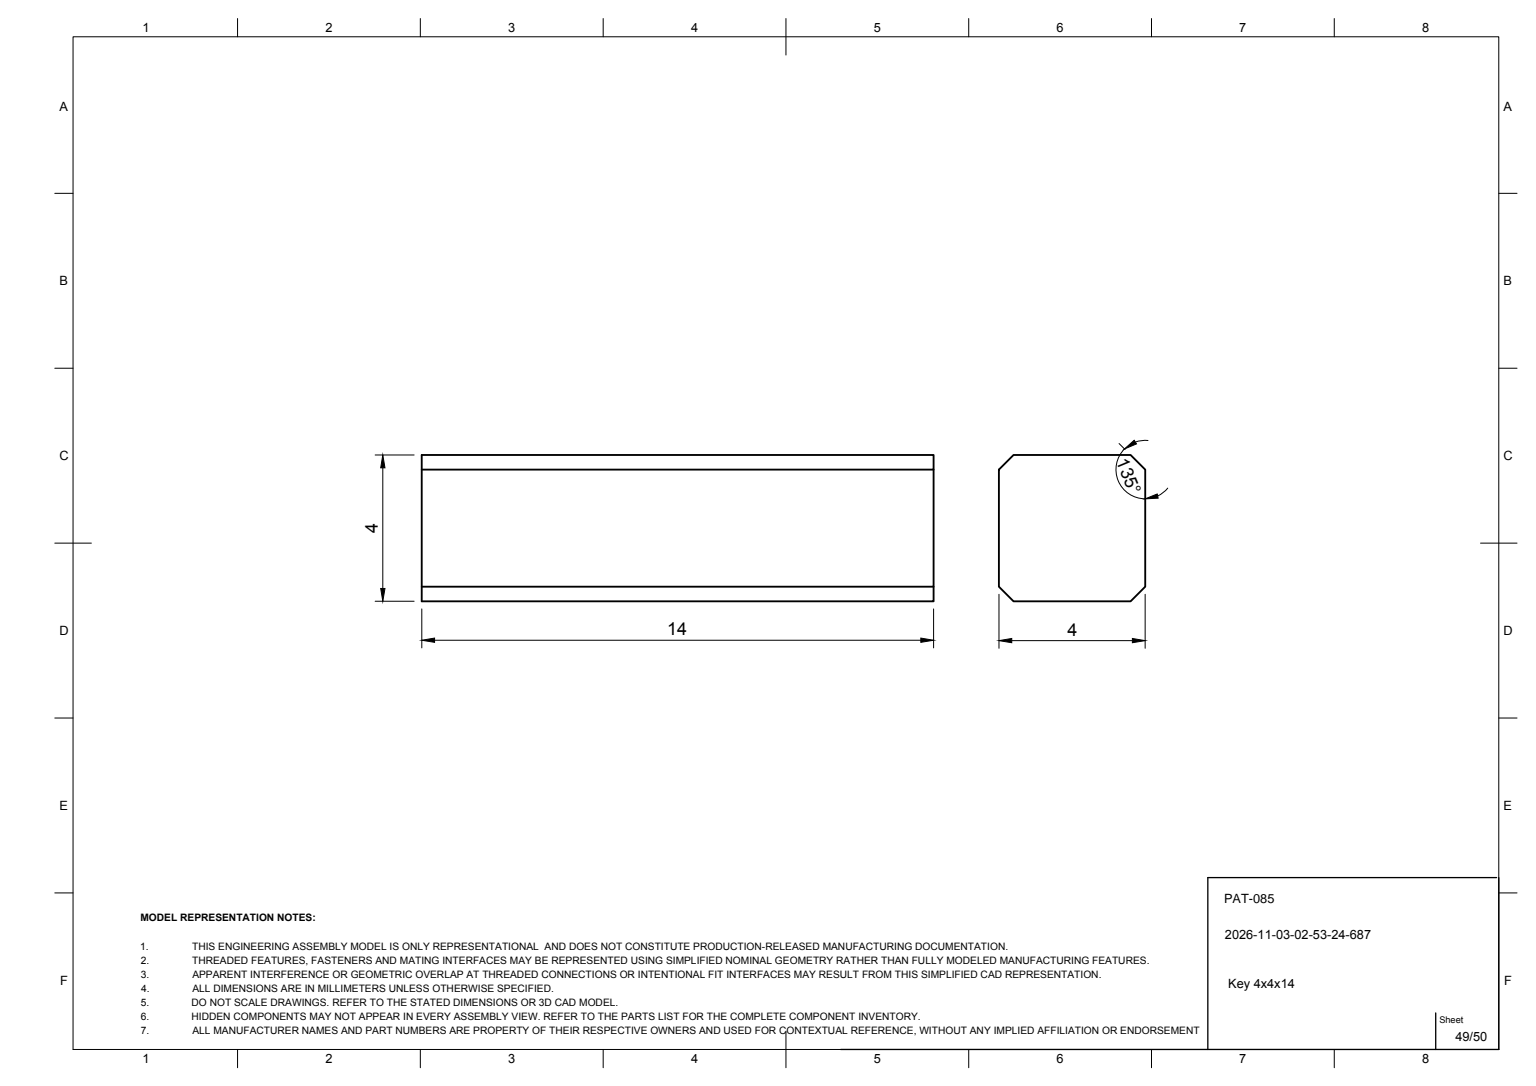
ISO-10303-21;
HEADER;
/* Generated by software containing ST-Developer
 * from STEP Tools, Inc. (www.steptools.com) 
 */

FILE_DESCRIPTION(
/* description */ ('Rack and pinion manual slide'),
/* implementation_level */ '2;1');

FILE_NAME(
/* name */ 'Key 4x4x14.step',
/* time_stamp */ '2026-10-28T03:22:49-07:00',
/* author */ (''),
/* organization */ (''),
/* preprocessor_version */ 'ST-DEVELOPER v20.2',
/* originating_system */ 'Autodesk Translation Framework v15.17.0.0',
/* authorisation */ '');

FILE_SCHEMA (('AUTOMOTIVE_DESIGN { 1 0 10303 214 3 1 1 }'));
ENDSEC;

DATA;
#10=MECHANICAL_DESIGN_GEOMETRIC_PRESENTATION_REPRESENTATION('',(#781),#34851);
#682=SHAPE_REPRESENTATION_RELATIONSHIP('SRR','None',#35121,#728);
#728=ADVANCED_BREP_SHAPE_REPRESENTATION('',(#830),#34846);
#781=STYLED_ITEM('',(#35411),#830);
#830=MANIFOLD_SOLID_BREP('Body1',#13805);
#1510=PLANE('',#15524);
#1511=PLANE('',#15525);
#1512=PLANE('',#15526);
#1513=PLANE('',#15527);
#1514=PLANE('',#15528);
#1515=PLANE('',#15529);
#1516=PLANE('',#15530);
#1517=PLANE('',#15531);
#1518=PLANE('',#15532);
#1519=PLANE('',#15533);
#2239=FACE_OUTER_BOUND('',#3184,.T.);
#2240=FACE_OUTER_BOUND('',#3185,.T.);
#2241=FACE_OUTER_BOUND('',#3186,.T.);
#2242=FACE_OUTER_BOUND('',#3187,.T.);
#2243=FACE_OUTER_BOUND('',#3188,.T.);
#2244=FACE_OUTER_BOUND('',#3189,.T.);
#2245=FACE_OUTER_BOUND('',#3190,.T.);
#2246=FACE_OUTER_BOUND('',#3191,.T.);
#2247=FACE_OUTER_BOUND('',#3192,.T.);
#2248=FACE_OUTER_BOUND('',#3193,.T.);
#3184=EDGE_LOOP('',(#12708,#12709,#12710,#12711,#12712,#12713,#12714,#12715));
#3185=EDGE_LOOP('',(#12716,#12717,#12718,#12719));
#3186=EDGE_LOOP('',(#12720,#12721,#12722,#12723));
#3187=EDGE_LOOP('',(#12724,#12725,#12726,#12727));
#3188=EDGE_LOOP('',(#12728,#12729,#12730,#12731));
#3189=EDGE_LOOP('',(#12732,#12733,#12734,#12735,#12736,#12737,#12738,#12739));
#3190=EDGE_LOOP('',(#12740,#12741,#12742,#12743));
#3191=EDGE_LOOP('',(#12744,#12745,#12746,#12747));
#3192=EDGE_LOOP('',(#12748,#12749,#12750,#12751));
#3193=EDGE_LOOP('',(#12752,#12753,#12754,#12755));
#4463=LINE('',#34575,#5754);
#4464=LINE('',#34577,#5755);
#4465=LINE('',#34579,#5756);
#4466=LINE('',#34581,#5757);
#4467=LINE('',#34583,#5758);
#4468=LINE('',#34585,#5759);
#4469=LINE('',#34587,#5760);
#4470=LINE('',#34588,#5761);
#4471=LINE('',#34591,#5762);
#4472=LINE('',#34593,#5763);
#4473=LINE('',#34594,#5764);
#4474=LINE('',#34597,#5765);
#4475=LINE('',#34598,#5766);
#4476=LINE('',#34601,#5767);
#4477=LINE('',#34602,#5768);
#4478=LINE('',#34605,#5769);
#4479=LINE('',#34606,#5770);
#4480=LINE('',#34609,#5771);
#4481=LINE('',#34611,#5772);
#4482=LINE('',#34613,#5773);
#4483=LINE('',#34614,#5774);
#4484=LINE('',#34616,#5775);
#4485=LINE('',#34618,#5776);
#4486=LINE('',#34620,#5777);
#5754=VECTOR('',#19255,1.);
#5755=VECTOR('',#19256,1.);
#5756=VECTOR('',#19257,1.);
#5757=VECTOR('',#19258,1.);
#5758=VECTOR('',#19259,1.);
#5759=VECTOR('',#19260,1.);
#5760=VECTOR('',#19261,1.);
#5761=VECTOR('',#19262,1.);
#5762=VECTOR('',#19265,1.);
#5763=VECTOR('',#19266,1.);
#5764=VECTOR('',#19267,1.);
#5765=VECTOR('',#19270,1.);
#5766=VECTOR('',#19271,1.);
#5767=VECTOR('',#19274,1.);
#5768=VECTOR('',#19275,1.);
#5769=VECTOR('',#19278,1.);
#5770=VECTOR('',#19279,1.);
#5771=VECTOR('',#19282,1.);
#5772=VECTOR('',#19283,1.);
#5773=VECTOR('',#19284,1.);
#5774=VECTOR('',#19285,1.);
#5775=VECTOR('',#19288,1.);
#5776=VECTOR('',#19291,1.);
#5777=VECTOR('',#19294,1.);
#7385=VERTEX_POINT('',#34573);
#7386=VERTEX_POINT('',#34574);
#7387=VERTEX_POINT('',#34576);
#7388=VERTEX_POINT('',#34578);
#7389=VERTEX_POINT('',#34580);
#7390=VERTEX_POINT('',#34582);
#7391=VERTEX_POINT('',#34584);
#7392=VERTEX_POINT('',#34586);
#7393=VERTEX_POINT('',#34590);
#7394=VERTEX_POINT('',#34592);
#7395=VERTEX_POINT('',#34596);
#7396=VERTEX_POINT('',#34600);
#7397=VERTEX_POINT('',#34604);
#7398=VERTEX_POINT('',#34608);
#7399=VERTEX_POINT('',#34610);
#7400=VERTEX_POINT('',#34612);
#9166=EDGE_CURVE('',#7385,#7386,#4463,.T.);
#9167=EDGE_CURVE('',#7387,#7385,#4464,.T.);
#9168=EDGE_CURVE('',#7388,#7387,#4465,.T.);
#9169=EDGE_CURVE('',#7389,#7388,#4466,.T.);
#9170=EDGE_CURVE('',#7390,#7389,#4467,.T.);
#9171=EDGE_CURVE('',#7391,#7390,#4468,.T.);
#9172=EDGE_CURVE('',#7392,#7391,#4469,.T.);
#9173=EDGE_CURVE('',#7386,#7392,#4470,.T.);
#9174=EDGE_CURVE('',#7389,#7393,#4471,.T.);
#9175=EDGE_CURVE('',#7393,#7394,#4472,.T.);
#9176=EDGE_CURVE('',#7394,#7390,#4473,.T.);
#9177=EDGE_CURVE('',#7395,#7388,#4474,.T.);
#9178=EDGE_CURVE('',#7395,#7393,#4475,.T.);
#9179=EDGE_CURVE('',#7387,#7396,#4476,.T.);
#9180=EDGE_CURVE('',#7396,#7395,#4477,.T.);
#9181=EDGE_CURVE('',#7397,#7385,#4478,.T.);
#9182=EDGE_CURVE('',#7397,#7396,#4479,.T.);
#9183=EDGE_CURVE('',#7398,#7397,#4480,.T.);
#9184=EDGE_CURVE('',#7399,#7398,#4481,.T.);
#9185=EDGE_CURVE('',#7400,#7399,#4482,.T.);
#9186=EDGE_CURVE('',#7394,#7400,#4483,.T.);
#9187=EDGE_CURVE('',#7386,#7398,#4484,.T.);
#9188=EDGE_CURVE('',#7399,#7392,#4485,.T.);
#9189=EDGE_CURVE('',#7391,#7400,#4486,.T.);
#12708=ORIENTED_EDGE('',*,*,#9166,.F.);
#12709=ORIENTED_EDGE('',*,*,#9167,.F.);
#12710=ORIENTED_EDGE('',*,*,#9168,.F.);
#12711=ORIENTED_EDGE('',*,*,#9169,.F.);
#12712=ORIENTED_EDGE('',*,*,#9170,.F.);
#12713=ORIENTED_EDGE('',*,*,#9171,.F.);
#12714=ORIENTED_EDGE('',*,*,#9172,.F.);
#12715=ORIENTED_EDGE('',*,*,#9173,.F.);
#12716=ORIENTED_EDGE('',*,*,#9170,.T.);
#12717=ORIENTED_EDGE('',*,*,#9174,.T.);
#12718=ORIENTED_EDGE('',*,*,#9175,.T.);
#12719=ORIENTED_EDGE('',*,*,#9176,.T.);
#12720=ORIENTED_EDGE('',*,*,#9169,.T.);
#12721=ORIENTED_EDGE('',*,*,#9177,.F.);
#12722=ORIENTED_EDGE('',*,*,#9178,.T.);
#12723=ORIENTED_EDGE('',*,*,#9174,.F.);
#12724=ORIENTED_EDGE('',*,*,#9168,.T.);
#12725=ORIENTED_EDGE('',*,*,#9179,.T.);
#12726=ORIENTED_EDGE('',*,*,#9180,.T.);
#12727=ORIENTED_EDGE('',*,*,#9177,.T.);
#12728=ORIENTED_EDGE('',*,*,#9167,.T.);
#12729=ORIENTED_EDGE('',*,*,#9181,.F.);
#12730=ORIENTED_EDGE('',*,*,#9182,.T.);
#12731=ORIENTED_EDGE('',*,*,#9179,.F.);
#12732=ORIENTED_EDGE('',*,*,#9175,.F.);
#12733=ORIENTED_EDGE('',*,*,#9178,.F.);
#12734=ORIENTED_EDGE('',*,*,#9180,.F.);
#12735=ORIENTED_EDGE('',*,*,#9182,.F.);
#12736=ORIENTED_EDGE('',*,*,#9183,.F.);
#12737=ORIENTED_EDGE('',*,*,#9184,.F.);
#12738=ORIENTED_EDGE('',*,*,#9185,.F.);
#12739=ORIENTED_EDGE('',*,*,#9186,.F.);
#12740=ORIENTED_EDGE('',*,*,#9166,.T.);
#12741=ORIENTED_EDGE('',*,*,#9187,.T.);
#12742=ORIENTED_EDGE('',*,*,#9183,.T.);
#12743=ORIENTED_EDGE('',*,*,#9181,.T.);
#12744=ORIENTED_EDGE('',*,*,#9173,.T.);
#12745=ORIENTED_EDGE('',*,*,#9188,.F.);
#12746=ORIENTED_EDGE('',*,*,#9184,.T.);
#12747=ORIENTED_EDGE('',*,*,#9187,.F.);
#12748=ORIENTED_EDGE('',*,*,#9172,.T.);
#12749=ORIENTED_EDGE('',*,*,#9189,.T.);
#12750=ORIENTED_EDGE('',*,*,#9185,.T.);
#12751=ORIENTED_EDGE('',*,*,#9188,.T.);
#12752=ORIENTED_EDGE('',*,*,#9171,.T.);
#12753=ORIENTED_EDGE('',*,*,#9176,.F.);
#12754=ORIENTED_EDGE('',*,*,#9186,.T.);
#12755=ORIENTED_EDGE('',*,*,#9189,.F.);
#13717=ADVANCED_FACE('',(#2239),#1510,.T.);
#13718=ADVANCED_FACE('',(#2240),#1511,.T.);
#13719=ADVANCED_FACE('',(#2241),#1512,.T.);
#13720=ADVANCED_FACE('',(#2242),#1513,.T.);
#13721=ADVANCED_FACE('',(#2243),#1514,.T.);
#13722=ADVANCED_FACE('',(#2244),#1515,.F.);
#13723=ADVANCED_FACE('',(#2245),#1516,.T.);
#13724=ADVANCED_FACE('',(#2246),#1517,.T.);
#13725=ADVANCED_FACE('',(#2247),#1518,.T.);
#13726=ADVANCED_FACE('',(#2248),#1519,.F.);
#13805=CLOSED_SHELL('',(#13717,#13718,#13719,#13720,#13721,#13722,#13723,
#13724,#13725,#13726));
#15523=AXIS2_PLACEMENT_3D('',#34571,#19251,#19252);
#15524=AXIS2_PLACEMENT_3D('',#34572,#19253,#19254);
#15525=AXIS2_PLACEMENT_3D('',#34589,#19263,#19264);
#15526=AXIS2_PLACEMENT_3D('',#34595,#19268,#19269);
#15527=AXIS2_PLACEMENT_3D('',#34599,#19272,#19273);
#15528=AXIS2_PLACEMENT_3D('',#34603,#19276,#19277);
#15529=AXIS2_PLACEMENT_3D('',#34607,#19280,#19281);
#15530=AXIS2_PLACEMENT_3D('',#34615,#19286,#19287);
#15531=AXIS2_PLACEMENT_3D('',#34617,#19289,#19290);
#15532=AXIS2_PLACEMENT_3D('',#34619,#19292,#19293);
#15533=AXIS2_PLACEMENT_3D('',#34621,#19295,#19296);
#19251=DIRECTION('axis',(0.,0.,1.));
#19252=DIRECTION('refdir',(1.,0.,0.));
#19253=DIRECTION('center_axis',(1.,0.,0.));
#19254=DIRECTION('ref_axis',(0.,0.,-1.));
#19255=DIRECTION('',(0.,0.707106781186547,-0.707106781186548));
#19256=DIRECTION('',(0.,1.,0.));
#19257=DIRECTION('',(0.,0.707106781186547,0.707106781186548));
#19258=DIRECTION('',(0.,0.,1.));
#19259=DIRECTION('',(0.,-0.707106781186548,0.707106781186548));
#19260=DIRECTION('',(0.,-1.,0.));
#19261=DIRECTION('',(0.,-0.707106781186548,-0.707106781186548));
#19262=DIRECTION('',(0.,0.,-1.));
#19263=DIRECTION('center_axis',(0.,-0.707106781186548,-0.707106781186548));
#19264=DIRECTION('ref_axis',(-1.,0.,0.));
#19265=DIRECTION('',(-1.,0.,0.));
#19266=DIRECTION('',(0.,0.707106781186548,-0.707106781186548));
#19267=DIRECTION('',(1.,0.,0.));
#19268=DIRECTION('center_axis',(0.,-1.,0.));
#19269=DIRECTION('ref_axis',(1.,0.,0.));
#19270=DIRECTION('',(1.,0.,0.));
#19271=DIRECTION('',(0.,0.,-1.));
#19272=DIRECTION('center_axis',(0.,-0.707106781186548,0.707106781186547));
#19273=DIRECTION('ref_axis',(1.,0.,0.));
#19274=DIRECTION('',(-1.,0.,0.));
#19275=DIRECTION('',(0.,-0.707106781186547,-0.707106781186548));
#19276=DIRECTION('center_axis',(0.,0.,1.));
#19277=DIRECTION('ref_axis',(1.,0.,0.));
#19278=DIRECTION('',(1.,0.,0.));
#19279=DIRECTION('',(0.,-1.,0.));
#19280=DIRECTION('center_axis',(1.,0.,0.));
#19281=DIRECTION('ref_axis',(0.,0.,-1.));
#19282=DIRECTION('',(0.,-0.707106781186547,0.707106781186548));
#19283=DIRECTION('',(0.,0.,1.));
#19284=DIRECTION('',(0.,0.707106781186548,0.707106781186548));
#19285=DIRECTION('',(0.,1.,0.));
#19286=DIRECTION('center_axis',(0.,0.707106781186548,0.707106781186547));
#19287=DIRECTION('ref_axis',(1.,0.,0.));
#19288=DIRECTION('',(-1.,0.,0.));
#19289=DIRECTION('center_axis',(0.,1.,0.));
#19290=DIRECTION('ref_axis',(-1.,0.,0.));
#19291=DIRECTION('',(1.,0.,0.));
#19292=DIRECTION('center_axis',(0.,0.707106781186548,-0.707106781186548));
#19293=DIRECTION('ref_axis',(-1.,0.,0.));
#19294=DIRECTION('',(-1.,0.,0.));
#19295=DIRECTION('center_axis',(0.,0.,1.));
#19296=DIRECTION('ref_axis',(1.,0.,0.));
#34571=CARTESIAN_POINT('',(0.,0.,0.));
#34572=CARTESIAN_POINT('Origin',(0.7,0.,0.25));
#34573=CARTESIAN_POINT('',(0.7,0.16,0.4));
#34574=CARTESIAN_POINT('',(0.7,0.2,0.36));
#34575=CARTESIAN_POINT('',(0.7,0.1675,0.3925));
#34576=CARTESIAN_POINT('',(0.7,-0.16,0.4));
#34577=CARTESIAN_POINT('',(0.7,0.,0.4));
#34578=CARTESIAN_POINT('',(0.7,-0.2,0.36));
#34579=CARTESIAN_POINT('',(0.7,-0.1675,0.3925));
#34580=CARTESIAN_POINT('',(0.7,-0.2,0.04));
#34581=CARTESIAN_POINT('',(0.7,-0.2,0.125));
#34582=CARTESIAN_POINT('',(0.7,-0.16,0.));
#34583=CARTESIAN_POINT('',(0.7,-0.1925,0.0325));
#34584=CARTESIAN_POINT('',(0.7,0.16,0.));
#34585=CARTESIAN_POINT('',(0.7,0.,0.));
#34586=CARTESIAN_POINT('',(0.7,0.2,0.04));
#34587=CARTESIAN_POINT('',(0.7,0.1925,0.0325));
#34588=CARTESIAN_POINT('',(0.7,0.2,0.125));
#34589=CARTESIAN_POINT('Origin',(-0.4,-0.18,0.02));
#34590=CARTESIAN_POINT('',(-0.7,-0.2,0.04));
#34591=CARTESIAN_POINT('',(-0.4,-0.2,0.04));
#34592=CARTESIAN_POINT('',(-0.7,-0.16,0.));
#34593=CARTESIAN_POINT('',(-0.7,-0.1925,0.0325));
#34594=CARTESIAN_POINT('',(-0.4,-0.16,0.));
#34595=CARTESIAN_POINT('Origin',(-0.8,-0.2,0.));
#34596=CARTESIAN_POINT('',(-0.7,-0.2,0.36));
#34597=CARTESIAN_POINT('',(-0.4,-0.2,0.36));
#34598=CARTESIAN_POINT('',(-0.7,-0.2,0.125));
#34599=CARTESIAN_POINT('Origin',(-0.4,-0.18,0.38));
#34600=CARTESIAN_POINT('',(-0.7,-0.16,0.4));
#34601=CARTESIAN_POINT('',(-0.4,-0.16,0.4));
#34602=CARTESIAN_POINT('',(-0.7,-0.1675,0.3925));
#34603=CARTESIAN_POINT('Origin',(0.,0.,0.4));
#34604=CARTESIAN_POINT('',(-0.7,0.16,0.4));
#34605=CARTESIAN_POINT('',(0.4,0.16,0.4));
#34606=CARTESIAN_POINT('',(-0.7,0.,0.4));
#34607=CARTESIAN_POINT('Origin',(-0.7,0.,0.25));
#34608=CARTESIAN_POINT('',(-0.7,0.2,0.36));
#34609=CARTESIAN_POINT('',(-0.7,0.1675,0.3925));
#34610=CARTESIAN_POINT('',(-0.7,0.2,0.04));
#34611=CARTESIAN_POINT('',(-0.7,0.2,0.125));
#34612=CARTESIAN_POINT('',(-0.7,0.16,0.));
#34613=CARTESIAN_POINT('',(-0.7,0.1925,0.0325));
#34614=CARTESIAN_POINT('',(-0.7,0.,0.));
#34615=CARTESIAN_POINT('Origin',(0.4,0.18,0.38));
#34616=CARTESIAN_POINT('',(0.4,0.2,0.36));
#34617=CARTESIAN_POINT('Origin',(0.8,0.2,0.));
#34618=CARTESIAN_POINT('',(0.4,0.2,0.04));
#34619=CARTESIAN_POINT('Origin',(0.4,0.18,0.02));
#34620=CARTESIAN_POINT('',(0.4,0.16,0.));
#34621=CARTESIAN_POINT('Origin',(0.,0.,0.));
#34792=UNCERTAINTY_MEASURE_WITH_UNIT(LENGTH_MEASURE(0.001),#34852,
'DISTANCE_ACCURACY_VALUE',
'Maximum model space distance between geometric entities at asserted c
onnectivities');
#34797=UNCERTAINTY_MEASURE_WITH_UNIT(LENGTH_MEASURE(0.001),#34852,
'DISTANCE_ACCURACY_VALUE',
'Maximum model space distance between geometric entities at asserted c
onnectivities');
#34846=(
GEOMETRIC_REPRESENTATION_CONTEXT(3)
GLOBAL_UNCERTAINTY_ASSIGNED_CONTEXT((#34792))
GLOBAL_UNIT_ASSIGNED_CONTEXT((#34852,#34854,#34855))
REPRESENTATION_CONTEXT('','3D')
);
#34851=(
GEOMETRIC_REPRESENTATION_CONTEXT(3)
GLOBAL_UNCERTAINTY_ASSIGNED_CONTEXT((#34797))
GLOBAL_UNIT_ASSIGNED_CONTEXT((#34852,#34854,#34855))
REPRESENTATION_CONTEXT('','3D')
);
#34852=(
LENGTH_UNIT()
NAMED_UNIT(*)
SI_UNIT(.CENTI.,.METRE.)
);
#34854=(
NAMED_UNIT(*)
PLANE_ANGLE_UNIT()
SI_UNIT($,.RADIAN.)
);
#34855=(
NAMED_UNIT(*)
SI_UNIT($,.STERADIAN.)
SOLID_ANGLE_UNIT()
);
#34904=SHAPE_DEFINITION_REPRESENTATION(#35047,#35121);
#35047=PRODUCT_DEFINITION_SHAPE('',$,#35175);
#35121=SHAPE_REPRESENTATION('',(#15523),#34846);
#35126=PRODUCT_DEFINITION_CONTEXT('part definition',#35287,'design');
#35175=PRODUCT_DEFINITION('Key 4x4x14','Key 4x4x14',#35228,#35126);
#35228=PRODUCT_DEFINITION_FORMATION('',$,#35337);
#35287=APPLICATION_CONTEXT(
'Core Data for Automotive Mechanical Design Process');
#35288=PRODUCT_CONTEXT('part definition',#35287,'mechanical');
#35337=PRODUCT('Key 4x4x14','Key 4x4x14','Key 4x4x14',(#35288));
#35405=COLOUR_RGB('Grey',0.48,0.52,0.57);
#35406=FILL_AREA_STYLE_COLOUR('',#35405);
#35407=FILL_AREA_STYLE('',(#35406));
#35408=SURFACE_STYLE_FILL_AREA(#35407);
#35409=SURFACE_SIDE_STYLE('',(#35408));
#35410=SURFACE_STYLE_USAGE(.BOTH.,#35409);
#35411=PRESENTATION_STYLE_ASSIGNMENT((#35410));
ENDSEC;
END-ISO-10303-21;
